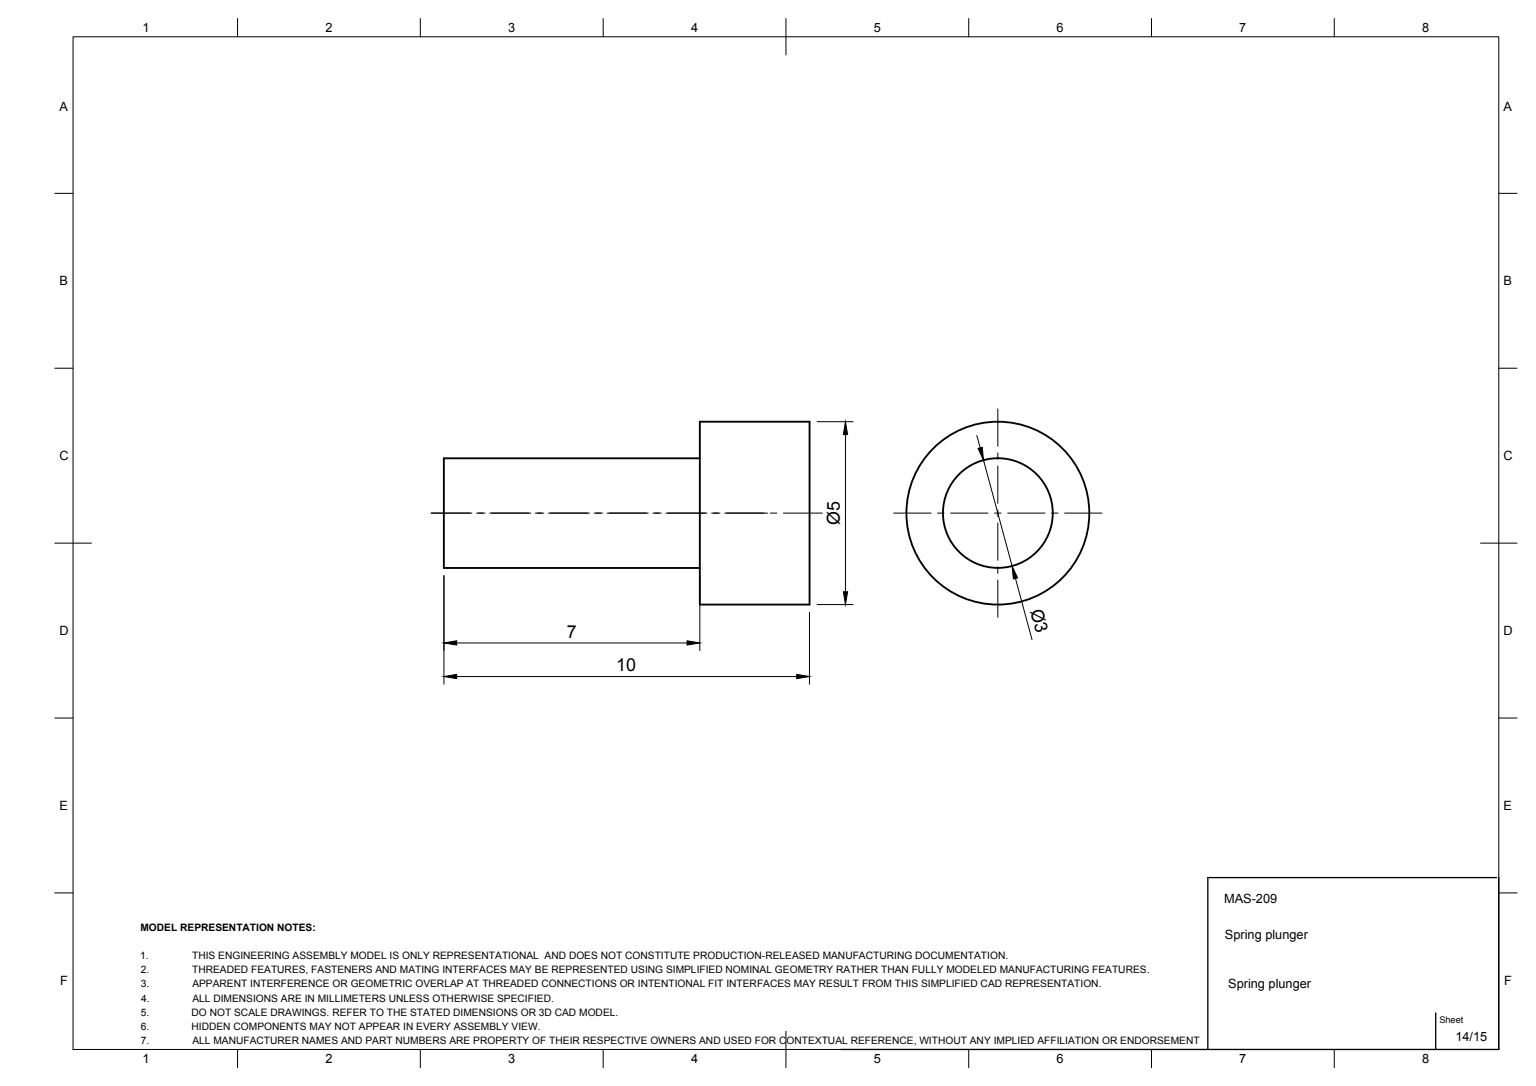
ISO-10303-21;
HEADER;
/* Generated by software containing ST-Developer
 * from STEP Tools, Inc. (www.steptools.com) 
 */

FILE_DESCRIPTION(
/* description */ ('Independent bearing-supported roller-ramp one-way clutch. Six logarit
hmic ramps with plain solid rollers, sprung guided plungers, native Co
il variants, removable shared keepers, rounded parallel key, shaft wit
h complete retaining lips, bronze journal/thrust support and bolted co
vers. Native rotor, roller planar/spin and plunger joints permit manua
l geometric engaged/released inspection. Automatic frictional torque s
witching/contact dynamics are not simulated; no capacity, hardness, fi
t, lubrication, speed, force or life rating. External input driver/cou
pling/anchors outside assembly.'),
/* implementation_level */ '2;1');

FILE_NAME(
/* name */ 'Spring plunger.step',
/* time_stamp */ '2026-11-08T07:04:38-08:00',
/* author */ (''),
/* organization */ (''),
/* preprocessor_version */ 'ST-DEVELOPER v20.2',
/* originating_system */ 'Autodesk Translation Framework v15.17.0.0',
/* authorisation */ '');

FILE_SCHEMA (('AUTOMOTIVE_DESIGN { 1 0 10303 214 3 1 1 }'));
ENDSEC;

DATA;
#10=MECHANICAL_DESIGN_GEOMETRIC_PRESENTATION_REPRESENTATION('',(#312),#99526);
#280=SHAPE_REPRESENTATION_RELATIONSHIP('SRR','None',#99637,#296);
#296=ADVANCED_BREP_SHAPE_REPRESENTATION('',(#328),#99522);
#312=STYLED_ITEM('',(#99723),#328);
#328=MANIFOLD_SOLID_BREP('Body1',#18282);
#436=FACE_BOUND('',#2686,.T.);
#589=PLANE('',#19633);
#590=PLANE('',#19638);
#591=PLANE('',#19641);
#1584=FACE_OUTER_BOUND('',#2685,.T.);
#1585=FACE_OUTER_BOUND('',#2687,.T.);
#1586=FACE_OUTER_BOUND('',#2688,.T.);
#1587=FACE_OUTER_BOUND('',#2689,.T.);
#1588=FACE_OUTER_BOUND('',#2690,.T.);
#2685=EDGE_LOOP('',(#16080));
#2686=EDGE_LOOP('',(#16081));
#2687=EDGE_LOOP('',(#16082,#16083,#16084,#16085));
#2688=EDGE_LOOP('',(#16086));
#2689=EDGE_LOOP('',(#16087,#16088,#16089,#16090));
#2690=EDGE_LOOP('',(#16091));
#3092=CIRCLE('',#19634,2.5);
#3093=CIRCLE('',#19635,1.5);
#3094=CIRCLE('',#19637,2.5);
#3095=CIRCLE('',#19640,1.5);
#5444=LINE('',#94930,#6348);
#5445=LINE('',#94934,#6349);
#6348=VECTOR('',#22963,2.5);
#6349=VECTOR('',#22968,1.5);
#8111=VERTEX_POINT('',#94923);
#8112=VERTEX_POINT('',#94925);
#8113=VERTEX_POINT('',#94928);
#8114=VERTEX_POINT('',#94933);
#10792=EDGE_CURVE('',#8111,#8111,#3092,.T.);
#10793=EDGE_CURVE('',#8112,#8112,#3093,.T.);
#10794=EDGE_CURVE('',#8113,#8113,#3094,.T.);
#10795=EDGE_CURVE('',#8113,#8111,#5444,.T.);
#10796=EDGE_CURVE('',#8112,#8114,#5445,.T.);
#10797=EDGE_CURVE('',#8114,#8114,#3095,.T.);
#16080=ORIENTED_EDGE('',*,*,#10792,.F.);
#16081=ORIENTED_EDGE('',*,*,#10793,.T.);
#16082=ORIENTED_EDGE('',*,*,#10794,.F.);
#16083=ORIENTED_EDGE('',*,*,#10795,.T.);
#16084=ORIENTED_EDGE('',*,*,#10792,.T.);
#16085=ORIENTED_EDGE('',*,*,#10795,.F.);
#16086=ORIENTED_EDGE('',*,*,#10794,.T.);
#16087=ORIENTED_EDGE('',*,*,#10793,.F.);
#16088=ORIENTED_EDGE('',*,*,#10796,.T.);
#16089=ORIENTED_EDGE('',*,*,#10797,.T.);
#16090=ORIENTED_EDGE('',*,*,#10796,.F.);
#16091=ORIENTED_EDGE('',*,*,#10797,.F.);
#17218=CYLINDRICAL_SURFACE('',#19636,2.5);
#17219=CYLINDRICAL_SURFACE('',#19639,1.5);
#18182=ADVANCED_FACE('',(#1584,#436),#589,.F.);
#18183=ADVANCED_FACE('',(#1585),#17218,.T.);
#18184=ADVANCED_FACE('',(#1586),#590,.T.);
#18185=ADVANCED_FACE('',(#1587),#17219,.T.);
#18186=ADVANCED_FACE('',(#1588),#591,.F.);
#18282=CLOSED_SHELL('',(#18182,#18183,#18184,#18185,#18186));
#19632=AXIS2_PLACEMENT_3D('',#94921,#22951,#22952);
#19633=AXIS2_PLACEMENT_3D('',#94922,#22953,#22954);
#19634=AXIS2_PLACEMENT_3D('',#94924,#22955,#22956);
#19635=AXIS2_PLACEMENT_3D('',#94926,#22957,#22958);
#19636=AXIS2_PLACEMENT_3D('',#94927,#22959,#22960);
#19637=AXIS2_PLACEMENT_3D('',#94929,#22961,#22962);
#19638=AXIS2_PLACEMENT_3D('',#94931,#22964,#22965);
#19639=AXIS2_PLACEMENT_3D('',#94932,#22966,#22967);
#19640=AXIS2_PLACEMENT_3D('',#94935,#22969,#22970);
#19641=AXIS2_PLACEMENT_3D('',#94936,#22971,#22972);
#22951=DIRECTION('axis',(0.,0.,1.));
#22952=DIRECTION('refdir',(1.,0.,0.));
#22953=DIRECTION('center_axis',(0.,0.,1.));
#22954=DIRECTION('ref_axis',(1.,0.,0.));
#22955=DIRECTION('center_axis',(0.,0.,1.));
#22956=DIRECTION('ref_axis',(1.,0.,0.));
#22957=DIRECTION('center_axis',(0.,0.,1.));
#22958=DIRECTION('ref_axis',(1.,0.,0.));
#22959=DIRECTION('center_axis',(0.,0.,1.));
#22960=DIRECTION('ref_axis',(1.,0.,0.));
#22961=DIRECTION('center_axis',(0.,0.,1.));
#22962=DIRECTION('ref_axis',(1.,0.,0.));
#22963=DIRECTION('',(0.,0.,-1.));
#22964=DIRECTION('center_axis',(0.,0.,1.));
#22965=DIRECTION('ref_axis',(1.,0.,0.));
#22966=DIRECTION('center_axis',(0.,0.,1.));
#22967=DIRECTION('ref_axis',(1.,0.,0.));
#22968=DIRECTION('',(0.,0.,-1.));
#22969=DIRECTION('center_axis',(0.,0.,1.));
#22970=DIRECTION('ref_axis',(1.,0.,0.));
#22971=DIRECTION('center_axis',(0.,0.,1.));
#22972=DIRECTION('ref_axis',(1.,0.,0.));
#94921=CARTESIAN_POINT('',(0.,0.,0.));
#94922=CARTESIAN_POINT('Origin',(0.,0.,6.));
#94923=CARTESIAN_POINT('',(-2.5,-3.06161699786838E-16,6.));
#94924=CARTESIAN_POINT('Origin',(0.,0.,6.));
#94925=CARTESIAN_POINT('',(-1.5,-1.83697019872103E-16,6.));
#94926=CARTESIAN_POINT('Origin',(0.,0.,6.));
#94927=CARTESIAN_POINT('Origin',(0.,0.,6.));
#94928=CARTESIAN_POINT('',(-2.5,-3.06161699786838E-16,9.));
#94929=CARTESIAN_POINT('Origin',(0.,0.,9.));
#94930=CARTESIAN_POINT('',(-2.5,-3.06161699786838E-16,6.));
#94931=CARTESIAN_POINT('Origin',(0.,0.,9.));
#94932=CARTESIAN_POINT('Origin',(0.,0.,-1.));
#94933=CARTESIAN_POINT('',(-1.5,-1.83697019872103E-16,-1.));
#94934=CARTESIAN_POINT('',(-1.5,-1.83697019872103E-16,-1.));
#94935=CARTESIAN_POINT('Origin',(0.,0.,-1.));
#94936=CARTESIAN_POINT('Origin',(0.,0.,-1.));
#99504=UNCERTAINTY_MEASURE_WITH_UNIT(LENGTH_MEASURE(0.01),#99527,
'DISTANCE_ACCURACY_VALUE',
'Maximum model space distance between geometric entities at asserted c
onnectivities');
#99508=UNCERTAINTY_MEASURE_WITH_UNIT(LENGTH_MEASURE(0.01),#99527,
'DISTANCE_ACCURACY_VALUE',
'Maximum model space distance between geometric entities at asserted c
onnectivities');
#99522=(
GEOMETRIC_REPRESENTATION_CONTEXT(3)
GLOBAL_UNCERTAINTY_ASSIGNED_CONTEXT((#99504))
GLOBAL_UNIT_ASSIGNED_CONTEXT((#99527,#99529,#99530))
REPRESENTATION_CONTEXT('','3D')
);
#99526=(
GEOMETRIC_REPRESENTATION_CONTEXT(3)
GLOBAL_UNCERTAINTY_ASSIGNED_CONTEXT((#99508))
GLOBAL_UNIT_ASSIGNED_CONTEXT((#99527,#99529,#99530))
REPRESENTATION_CONTEXT('','3D')
);
#99527=(
LENGTH_UNIT()
NAMED_UNIT(*)
SI_UNIT(.MILLI.,.METRE.)
);
#99529=(
NAMED_UNIT(*)
PLANE_ANGLE_UNIT()
SI_UNIT($,.RADIAN.)
);
#99530=(
NAMED_UNIT(*)
SI_UNIT($,.STERADIAN.)
SOLID_ANGLE_UNIT()
);
#99544=SHAPE_DEFINITION_REPRESENTATION(#99561,#99637);
#99561=PRODUCT_DEFINITION_SHAPE('',$,#99655);
#99637=SHAPE_REPRESENTATION('',(#19632),#99522);
#99641=PRODUCT_DEFINITION_CONTEXT('part definition',#99694,'design');
#99655=PRODUCT_DEFINITION('Spring plunger','Spring plunger',#99672,#99641);
#99672=PRODUCT_DEFINITION_FORMATION('',$,#99709);
#99694=APPLICATION_CONTEXT(
'Core Data for Automotive Mechanical Design Process');
#99695=PRODUCT_CONTEXT('part definition',#99694,'mechanical');
#99709=PRODUCT('Spring plunger','Spring plunger',$,(#99695));
#99723=PRESENTATION_STYLE_ASSIGNMENT((#99736));
#99736=SURFACE_STYLE_USAGE(.BOTH.,#99749);
#99749=SURFACE_SIDE_STYLE('',(#99762));
#99762=SURFACE_STYLE_FILL_AREA(#99775);
#99775=FILL_AREA_STYLE('Plunger light gray',(#99788));
#99788=FILL_AREA_STYLE_COLOUR('Plunger light gray',#99801);
#99801=COLOUR_RGB('Plunger light gray',0.725490196078431,0.752941176470588,
0.792156862745098);
ENDSEC;
END-ISO-10303-21;
